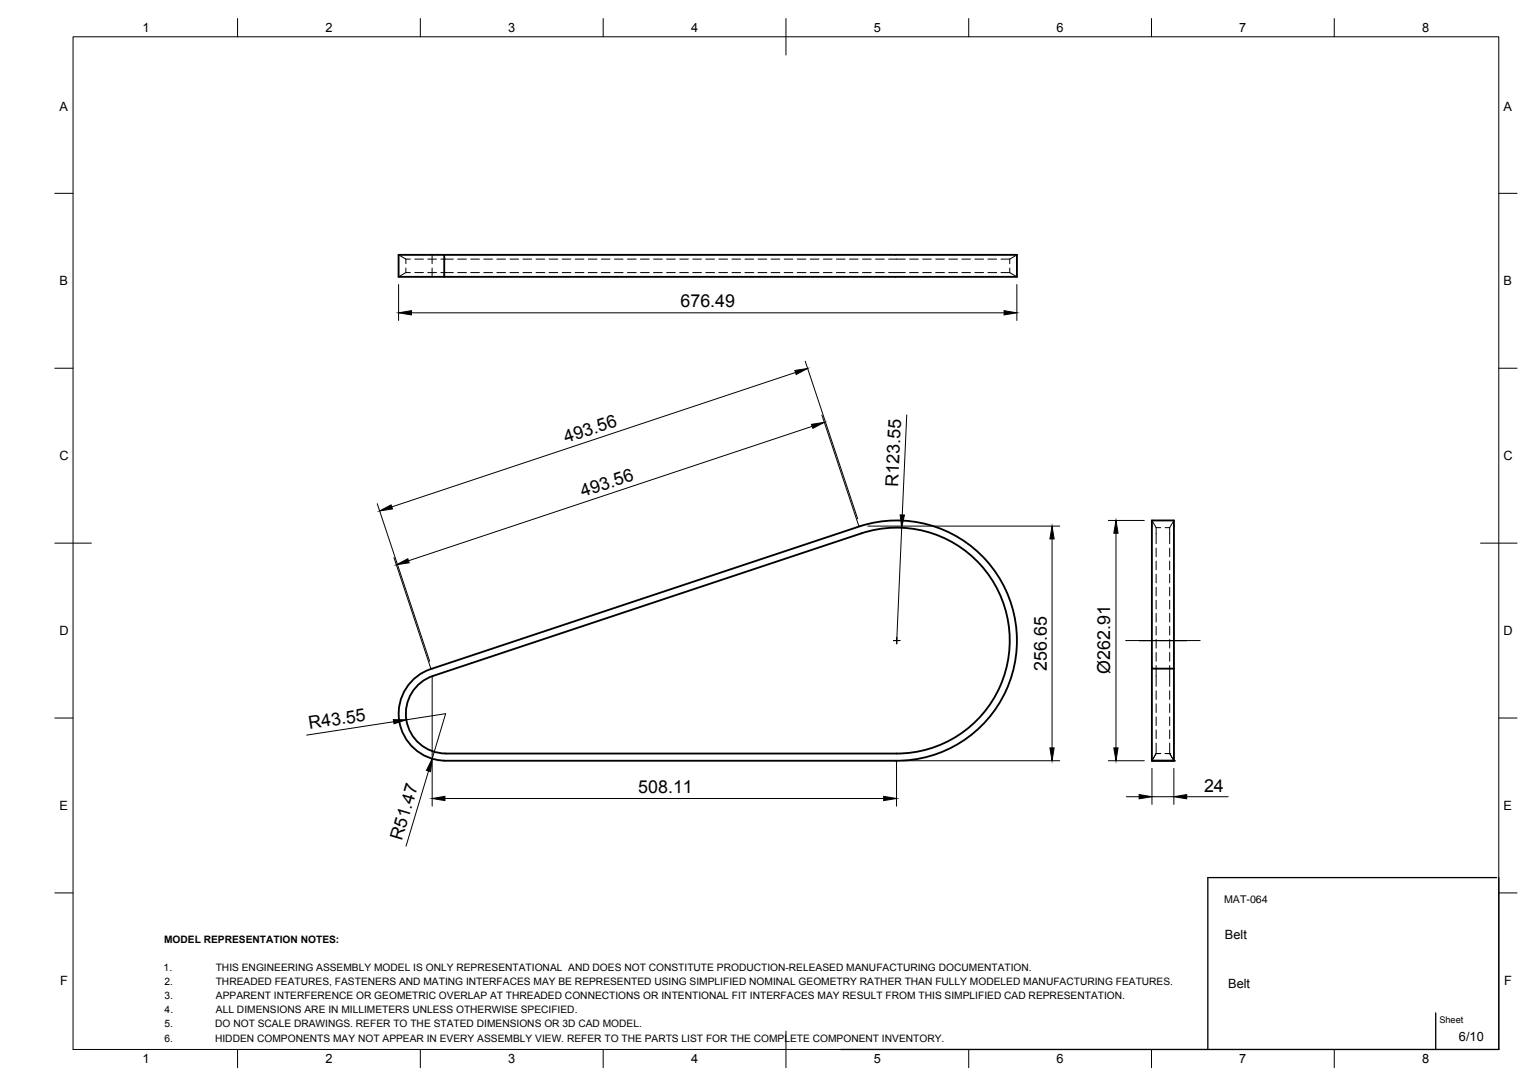
ISO-10303-21;
HEADER;
/* Generated by software containing ST-Developer
 * from STEP Tools, Inc. (www.steptools.com) 
 */

FILE_DESCRIPTION(
/* description */ (''),
/* implementation_level */ '2;1');

FILE_NAME(
/* name */ 
'Belt.step',
/* time_stamp */ '2026-10-24T12:42:14-07:00',
/* author */ (''),
/* organization */ (''),
/* preprocessor_version */ 'ST-DEVELOPER v20.2',
/* originating_system */ 'Autodesk Translation Framework v15.15.0.0',
/* authorisation */ '');

FILE_SCHEMA (('AUTOMOTIVE_DESIGN { 1 0 10303 214 3 1 1 }'));
ENDSEC;

DATA;
#10=MECHANICAL_DESIGN_GEOMETRIC_PRESENTATION_REPRESENTATION('',(#71),#6789);
#11=(
BOUNDED_SURFACE()
B_SPLINE_SURFACE(1,3,((#6689,#6690,#6691,#6692),(#6693,#6694,#6695,#6696)),
 .UNSPECIFIED.,.F.,.F.,.F.)
B_SPLINE_SURFACE_WITH_KNOTS((2,2),(4,4),(0.,1.),(0.,1.),.UNSPECIFIED.)
GEOMETRIC_REPRESENTATION_ITEM()
RATIONAL_B_SPLINE_SURFACE(((1.,0.44,0.44,1.),(1.,0.44,0.44,1.)))
REPRESENTATION_ITEM('')
SURFACE()
);
#12=(
BOUNDED_SURFACE()
B_SPLINE_SURFACE(1,3,((#6704,#6705,#6706,#6707),(#6708,#6709,#6710,#6711)),
 .UNSPECIFIED.,.F.,.F.,.F.)
B_SPLINE_SURFACE_WITH_KNOTS((2,2),(4,4),(0.,1.),(0.,1.),.UNSPECIFIED.)
GEOMETRIC_REPRESENTATION_ITEM()
RATIONAL_B_SPLINE_SURFACE(((1.,0.44,0.44,1.),(1.,0.44,0.44,1.)))
REPRESENTATION_ITEM('')
SURFACE()
);
#13=(
BOUNDED_SURFACE()
B_SPLINE_SURFACE(1,3,((#6733,#6734,#6735,#6736,#6737,#6738,#6739),(#6740,
#6741,#6742,#6743,#6744,#6745,#6746)),.UNSPECIFIED.,.F.,.F.,.F.)
B_SPLINE_SURFACE_WITH_KNOTS((2,2),(4,3,4),(0.,1.),(0.,0.5,1.),
 .UNSPECIFIED.)
GEOMETRIC_REPRESENTATION_ITEM()
RATIONAL_B_SPLINE_SURFACE(((1.,0.765382713227191,0.765382713227191,1.,0.765382713227191,
0.765382713227191,1.),(1.,0.765382713227191,0.765382713227191,1.,0.765382713227191,
0.765382713227191,1.)))
REPRESENTATION_ITEM('')
SURFACE()
);
#14=(
BOUNDED_SURFACE()
B_SPLINE_SURFACE(1,3,((#6750,#6751,#6752,#6753,#6754,#6755,#6756),(#6757,
#6758,#6759,#6760,#6761,#6762,#6763)),.UNSPECIFIED.,.F.,.F.,.F.)
B_SPLINE_SURFACE_WITH_KNOTS((2,2),(4,3,4),(0.,1.),(0.,0.5,1.),
 .UNSPECIFIED.)
GEOMETRIC_REPRESENTATION_ITEM()
RATIONAL_B_SPLINE_SURFACE(((1.,0.765382713227191,0.765382713227191,1.,0.765382713227191,
0.765382713227191,1.),(1.,0.765382713227191,0.765382713227191,1.,0.765382713227191,
0.765382713227191,1.)))
REPRESENTATION_ITEM('')
SURFACE()
);
#59=SHAPE_REPRESENTATION_RELATIONSHIP('SRR','None',#6826,#65);
#65=ADVANCED_BREP_SHAPE_REPRESENTATION('',(#77),#6788);
#71=STYLED_ITEM('',(#6863),#77);
#77=MANIFOLD_SOLID_BREP('Belt',#3966);
#181=CYLINDRICAL_SURFACE('',#4409,51.471200702168);
#182=CYLINDRICAL_SURFACE('',#4413,43.5522017822105);
#183=CYLINDRICAL_SURFACE('',#4419,131.457333002004);
#184=CYLINDRICAL_SURFACE('',#4423,123.55173167544);
#386=CIRCLE('',#4410,51.471200702168);
#387=CIRCLE('',#4411,51.471200702168);
#388=CIRCLE('',#4412,43.5522017822105);
#389=CIRCLE('',#4414,43.5522017822105);
#390=CIRCLE('',#4420,131.457333002004);
#391=CIRCLE('',#4421,131.457333002004);
#392=CIRCLE('',#4422,123.55173167544);
#393=CIRCLE('',#4424,123.55173167544);
#595=FACE_OUTER_BOUND('',#869,.T.);
#596=FACE_OUTER_BOUND('',#870,.T.);
#597=FACE_OUTER_BOUND('',#871,.T.);
#598=FACE_OUTER_BOUND('',#872,.T.);
#599=FACE_OUTER_BOUND('',#873,.T.);
#600=FACE_OUTER_BOUND('',#874,.T.);
#601=FACE_OUTER_BOUND('',#875,.T.);
#602=FACE_OUTER_BOUND('',#876,.T.);
#603=FACE_OUTER_BOUND('',#877,.T.);
#604=FACE_OUTER_BOUND('',#878,.T.);
#605=FACE_OUTER_BOUND('',#879,.T.);
#606=FACE_OUTER_BOUND('',#880,.T.);
#607=FACE_OUTER_BOUND('',#881,.T.);
#608=FACE_OUTER_BOUND('',#882,.T.);
#609=FACE_OUTER_BOUND('',#883,.T.);
#610=FACE_OUTER_BOUND('',#884,.T.);
#869=EDGE_LOOP('',(#3561,#3562,#3563,#3564));
#870=EDGE_LOOP('',(#3565,#3566,#3567,#3568));
#871=EDGE_LOOP('',(#3569,#3570,#3571,#3572));
#872=EDGE_LOOP('',(#3573,#3574,#3575,#3576));
#873=EDGE_LOOP('',(#3577,#3578,#3579,#3580));
#874=EDGE_LOOP('',(#3581,#3582,#3583,#3584));
#875=EDGE_LOOP('',(#3585,#3586,#3587,#3588));
#876=EDGE_LOOP('',(#3589,#3590,#3591,#3592));
#877=EDGE_LOOP('',(#3593,#3594,#3595,#3596));
#878=EDGE_LOOP('',(#3597,#3598,#3599,#3600));
#879=EDGE_LOOP('',(#3601,#3602,#3603,#3604));
#880=EDGE_LOOP('',(#3605,#3606,#3607,#3608));
#881=EDGE_LOOP('',(#3609,#3610,#3611,#3612));
#882=EDGE_LOOP('',(#3613,#3614,#3615,#3616));
#883=EDGE_LOOP('',(#3617,#3618,#3619,#3620));
#884=EDGE_LOOP('',(#3621,#3622,#3623,#3624));
#1239=LINE('',#6665,#1617);
#1240=LINE('',#6667,#1618);
#1241=LINE('',#6669,#1619);
#1242=LINE('',#6670,#1620);
#1243=LINE('',#6674,#1621);
#1244=LINE('',#6675,#1622);
#1245=LINE('',#6676,#1623);
#1246=LINE('',#6680,#1624);
#1247=LINE('',#6681,#1625);
#1248=LINE('',#6682,#1626);
#1249=LINE('',#6687,#1627);
#1250=LINE('',#6699,#1628);
#1251=LINE('',#6703,#1629);
#1252=LINE('',#6712,#1630);
#1253=LINE('',#6713,#1631);
#1254=LINE('',#6716,#1632);
#1255=LINE('',#6718,#1633);
#1256=LINE('',#6719,#1634);
#1257=LINE('',#6722,#1635);
#1258=LINE('',#6723,#1636);
#1259=LINE('',#6726,#1637);
#1260=LINE('',#6727,#1638);
#1261=LINE('',#6729,#1639);
#1262=LINE('',#6764,#1640);
#1617=VECTOR('',#5532,493.558507170122);
#1618=VECTOR('',#5533,24.);
#1619=VECTOR('',#5534,493.558507170122);
#1620=VECTOR('',#5535,24.);
#1621=VECTOR('',#5538,493.558507170122);
#1622=VECTOR('',#5539,9.23760430703403);
#1623=VECTOR('',#5540,9.23760430703403);
#1624=VECTOR('',#5543,493.558507170122);
#1625=VECTOR('',#5544,14.762395692966);
#1626=VECTOR('',#5545,14.762395692966);
#1627=VECTOR('',#5550,24.);
#1628=VECTOR('',#5555,9.23760430703401);
#1629=VECTOR('',#5560,14.762395692966);
#1630=VECTOR('',#5561,9.237604307034);
#1631=VECTOR('',#5562,9.23760430703398);
#1632=VECTOR('',#5565,493.558507170122);
#1633=VECTOR('',#5566,24.);
#1634=VECTOR('',#5567,493.558507170122);
#1635=VECTOR('',#5570,493.558507170122);
#1636=VECTOR('',#5571,9.23760430703404);
#1637=VECTOR('',#5574,493.558507170122);
#1638=VECTOR('',#5575,14.762395692966);
#1639=VECTOR('',#5578,9.237604307034);
#1640=VECTOR('',#5591,9.23760430703399);
#1971=VERTEX_POINT('',#6663);
#1972=VERTEX_POINT('',#6664);
#1973=VERTEX_POINT('',#6666);
#1974=VERTEX_POINT('',#6668);
#1975=VERTEX_POINT('',#6672);
#1976=VERTEX_POINT('',#6673);
#1977=VERTEX_POINT('',#6678);
#1978=VERTEX_POINT('',#6679);
#1979=VERTEX_POINT('',#6684);
#1980=VERTEX_POINT('',#6686);
#1981=VERTEX_POINT('',#6697);
#1982=VERTEX_POINT('',#6701);
#1983=VERTEX_POINT('',#6715);
#1984=VERTEX_POINT('',#6717);
#1985=VERTEX_POINT('',#6721);
#1986=VERTEX_POINT('',#6725);
#2501=EDGE_CURVE('',#1971,#1972,#1239,.T.);
#2502=EDGE_CURVE('',#1971,#1973,#1240,.T.);
#2503=EDGE_CURVE('',#1973,#1974,#1241,.T.);
#2504=EDGE_CURVE('',#1972,#1974,#1242,.T.);
#2505=EDGE_CURVE('',#1975,#1976,#1243,.T.);
#2506=EDGE_CURVE('',#1975,#1971,#1244,.T.);
#2507=EDGE_CURVE('',#1976,#1972,#1245,.T.);
#2508=EDGE_CURVE('',#1977,#1978,#1246,.T.);
#2509=EDGE_CURVE('',#1977,#1975,#1247,.T.);
#2510=EDGE_CURVE('',#1978,#1976,#1248,.T.);
#2511=EDGE_CURVE('',#1979,#1971,#386,.T.);
#2512=EDGE_CURVE('',#1979,#1980,#1249,.T.);
#2513=EDGE_CURVE('',#1980,#1973,#387,.T.);
#2514=EDGE_CURVE('',#1981,#1975,#388,.T.);
#2515=EDGE_CURVE('',#1981,#1979,#1250,.T.);
#2516=EDGE_CURVE('',#1982,#1977,#389,.T.);
#2517=EDGE_CURVE('',#1982,#1981,#1251,.T.);
#2518=EDGE_CURVE('',#1973,#1977,#1252,.T.);
#2519=EDGE_CURVE('',#1980,#1982,#1253,.T.);
#2520=EDGE_CURVE('',#1983,#1979,#1254,.T.);
#2521=EDGE_CURVE('',#1983,#1984,#1255,.T.);
#2522=EDGE_CURVE('',#1984,#1980,#1256,.T.);
#2523=EDGE_CURVE('',#1985,#1981,#1257,.T.);
#2524=EDGE_CURVE('',#1985,#1983,#1258,.T.);
#2525=EDGE_CURVE('',#1986,#1982,#1259,.T.);
#2526=EDGE_CURVE('',#1986,#1985,#1260,.T.);
#2527=EDGE_CURVE('',#1984,#1986,#1261,.T.);
#2528=EDGE_CURVE('',#1972,#1983,#390,.T.);
#2529=EDGE_CURVE('',#1974,#1984,#391,.T.);
#2530=EDGE_CURVE('',#1976,#1985,#392,.T.);
#2531=EDGE_CURVE('',#1978,#1986,#393,.T.);
#2532=EDGE_CURVE('',#1974,#1978,#1262,.T.);
#3561=ORIENTED_EDGE('',*,*,#2501,.F.);
#3562=ORIENTED_EDGE('',*,*,#2502,.T.);
#3563=ORIENTED_EDGE('',*,*,#2503,.T.);
#3564=ORIENTED_EDGE('',*,*,#2504,.F.);
#3565=ORIENTED_EDGE('',*,*,#2505,.F.);
#3566=ORIENTED_EDGE('',*,*,#2506,.T.);
#3567=ORIENTED_EDGE('',*,*,#2501,.T.);
#3568=ORIENTED_EDGE('',*,*,#2507,.F.);
#3569=ORIENTED_EDGE('',*,*,#2508,.F.);
#3570=ORIENTED_EDGE('',*,*,#2509,.T.);
#3571=ORIENTED_EDGE('',*,*,#2505,.T.);
#3572=ORIENTED_EDGE('',*,*,#2510,.F.);
#3573=ORIENTED_EDGE('',*,*,#2502,.F.);
#3574=ORIENTED_EDGE('',*,*,#2511,.F.);
#3575=ORIENTED_EDGE('',*,*,#2512,.T.);
#3576=ORIENTED_EDGE('',*,*,#2513,.T.);
#3577=ORIENTED_EDGE('',*,*,#2511,.T.);
#3578=ORIENTED_EDGE('',*,*,#2506,.F.);
#3579=ORIENTED_EDGE('',*,*,#2514,.F.);
#3580=ORIENTED_EDGE('',*,*,#2515,.T.);
#3581=ORIENTED_EDGE('',*,*,#2514,.T.);
#3582=ORIENTED_EDGE('',*,*,#2509,.F.);
#3583=ORIENTED_EDGE('',*,*,#2516,.F.);
#3584=ORIENTED_EDGE('',*,*,#2517,.T.);
#3585=ORIENTED_EDGE('',*,*,#2516,.T.);
#3586=ORIENTED_EDGE('',*,*,#2518,.F.);
#3587=ORIENTED_EDGE('',*,*,#2513,.F.);
#3588=ORIENTED_EDGE('',*,*,#2519,.T.);
#3589=ORIENTED_EDGE('',*,*,#2512,.F.);
#3590=ORIENTED_EDGE('',*,*,#2520,.F.);
#3591=ORIENTED_EDGE('',*,*,#2521,.T.);
#3592=ORIENTED_EDGE('',*,*,#2522,.T.);
#3593=ORIENTED_EDGE('',*,*,#2520,.T.);
#3594=ORIENTED_EDGE('',*,*,#2515,.F.);
#3595=ORIENTED_EDGE('',*,*,#2523,.F.);
#3596=ORIENTED_EDGE('',*,*,#2524,.T.);
#3597=ORIENTED_EDGE('',*,*,#2523,.T.);
#3598=ORIENTED_EDGE('',*,*,#2517,.F.);
#3599=ORIENTED_EDGE('',*,*,#2525,.F.);
#3600=ORIENTED_EDGE('',*,*,#2526,.T.);
#3601=ORIENTED_EDGE('',*,*,#2525,.T.);
#3602=ORIENTED_EDGE('',*,*,#2519,.F.);
#3603=ORIENTED_EDGE('',*,*,#2522,.F.);
#3604=ORIENTED_EDGE('',*,*,#2527,.T.);
#3605=ORIENTED_EDGE('',*,*,#2521,.F.);
#3606=ORIENTED_EDGE('',*,*,#2528,.F.);
#3607=ORIENTED_EDGE('',*,*,#2504,.T.);
#3608=ORIENTED_EDGE('',*,*,#2529,.T.);
#3609=ORIENTED_EDGE('',*,*,#2528,.T.);
#3610=ORIENTED_EDGE('',*,*,#2524,.F.);
#3611=ORIENTED_EDGE('',*,*,#2530,.F.);
#3612=ORIENTED_EDGE('',*,*,#2507,.T.);
#3613=ORIENTED_EDGE('',*,*,#2530,.T.);
#3614=ORIENTED_EDGE('',*,*,#2526,.F.);
#3615=ORIENTED_EDGE('',*,*,#2531,.F.);
#3616=ORIENTED_EDGE('',*,*,#2510,.T.);
#3617=ORIENTED_EDGE('',*,*,#2531,.T.);
#3618=ORIENTED_EDGE('',*,*,#2527,.F.);
#3619=ORIENTED_EDGE('',*,*,#2529,.F.);
#3620=ORIENTED_EDGE('',*,*,#2532,.T.);
#3621=ORIENTED_EDGE('',*,*,#2518,.T.);
#3622=ORIENTED_EDGE('',*,*,#2508,.T.);
#3623=ORIENTED_EDGE('',*,*,#2532,.F.);
#3624=ORIENTED_EDGE('',*,*,#2503,.F.);
#3736=PLANE('',#4406);
#3737=PLANE('',#4407);
#3738=PLANE('',#4408);
#3739=PLANE('',#4415);
#3740=PLANE('',#4416);
#3741=PLANE('',#4417);
#3742=PLANE('',#4418);
#3743=PLANE('',#4425);
#3945=ADVANCED_FACE('',(#595),#3736,.T.);
#3946=ADVANCED_FACE('',(#596),#3737,.T.);
#3947=ADVANCED_FACE('',(#597),#3738,.T.);
#3948=ADVANCED_FACE('',(#598),#181,.T.);
#3949=ADVANCED_FACE('',(#599),#11,.T.);
#3950=ADVANCED_FACE('',(#600),#182,.F.);
#3951=ADVANCED_FACE('',(#601),#12,.T.);
#3952=ADVANCED_FACE('',(#602),#3739,.T.);
#3953=ADVANCED_FACE('',(#603),#3740,.T.);
#3954=ADVANCED_FACE('',(#604),#3741,.T.);
#3955=ADVANCED_FACE('',(#605),#3742,.T.);
#3956=ADVANCED_FACE('',(#606),#183,.T.);
#3957=ADVANCED_FACE('',(#607),#13,.T.);
#3958=ADVANCED_FACE('',(#608),#184,.F.);
#3959=ADVANCED_FACE('',(#609),#14,.T.);
#3960=ADVANCED_FACE('',(#610),#3743,.T.);
#3966=CLOSED_SHELL('',(#3945,#3946,#3947,#3948,#3949,#3950,#3951,#3952,
#3953,#3954,#3955,#3956,#3957,#3958,#3959,#3960));
#4405=AXIS2_PLACEMENT_3D('',#6661,#5528,#5529);
#4406=AXIS2_PLACEMENT_3D('',#6662,#5530,#5531);
#4407=AXIS2_PLACEMENT_3D('',#6671,#5536,#5537);
#4408=AXIS2_PLACEMENT_3D('',#6677,#5541,#5542);
#4409=AXIS2_PLACEMENT_3D('',#6683,#5546,#5547);
#4410=AXIS2_PLACEMENT_3D('',#6685,#5548,#5549);
#4411=AXIS2_PLACEMENT_3D('',#6688,#5551,#5552);
#4412=AXIS2_PLACEMENT_3D('',#6698,#5553,#5554);
#4413=AXIS2_PLACEMENT_3D('',#6700,#5556,#5557);
#4414=AXIS2_PLACEMENT_3D('',#6702,#5558,#5559);
#4415=AXIS2_PLACEMENT_3D('',#6714,#5563,#5564);
#4416=AXIS2_PLACEMENT_3D('',#6720,#5568,#5569);
#4417=AXIS2_PLACEMENT_3D('',#6724,#5572,#5573);
#4418=AXIS2_PLACEMENT_3D('',#6728,#5576,#5577);
#4419=AXIS2_PLACEMENT_3D('',#6730,#5579,#5580);
#4420=AXIS2_PLACEMENT_3D('',#6731,#5581,#5582);
#4421=AXIS2_PLACEMENT_3D('',#6732,#5583,#5584);
#4422=AXIS2_PLACEMENT_3D('',#6747,#5585,#5586);
#4423=AXIS2_PLACEMENT_3D('',#6748,#5587,#5588);
#4424=AXIS2_PLACEMENT_3D('',#6749,#5589,#5590);
#4425=AXIS2_PLACEMENT_3D('',#6765,#5592,#5593);
#5528=DIRECTION('axis',(0.,0.,1.));
#5529=DIRECTION('refdir',(1.,0.,0.));
#5530=DIRECTION('center_axis',(-0.159999999999998,0.987117014340246,0.));
#5531=DIRECTION('ref_axis',(0.,0.,1.));
#5532=DIRECTION('',(0.987117014340246,0.159999999999998,0.));
#5533=DIRECTION('',(0.,0.,1.));
#5534=DIRECTION('',(0.987117014340246,0.159999999999998,0.));
#5535=DIRECTION('',(0.,0.,1.));
#5536=DIRECTION('center_axis',(0.0807792391722015,-0.498366008702133,-0.863195247837398));
#5537=DIRECTION('ref_axis',(-0.995649789053195,0.,-0.0931745542427157));
#5538=DIRECTION('',(0.987117014340246,0.159999999999998,0.));
#5539=DIRECTION('',(0.,0.866025403784436,-0.500000000000004));
#5540=DIRECTION('',(0.,0.866025403784436,-0.500000000000004));
#5541=DIRECTION('center_axis',(0.159999999999998,-0.987117014340246,0.));
#5542=DIRECTION('ref_axis',(0.,0.,-1.));
#5543=DIRECTION('',(0.987117014340246,0.159999999999998,0.));
#5544=DIRECTION('',(0.,0.,-1.));
#5545=DIRECTION('',(0.,0.,-1.));
#5546=DIRECTION('center_axis',(0.,0.,-1.));
#5547=DIRECTION('ref_axis',(-1.,0.,0.));
#5548=DIRECTION('center_axis',(0.,0.,-1.));
#5549=DIRECTION('ref_axis',(-0.189299873786385,-0.98191932346016,0.));
#5550=DIRECTION('',(0.,0.,1.));
#5551=DIRECTION('center_axis',(0.,0.,-1.));
#5552=DIRECTION('ref_axis',(-0.189299873786385,-0.98191932346016,0.));
#5553=DIRECTION('center_axis',(0.,0.,-1.));
#5554=DIRECTION('ref_axis',(-0.1656970702866,-0.986176698618679,0.));
#5555=DIRECTION('',(-0.273557891496469,-0.821684903110675,-0.500000000000006));
#5556=DIRECTION('center_axis',(0.,0.,-1.));
#5557=DIRECTION('ref_axis',(-1.,0.,0.));
#5558=DIRECTION('center_axis',(0.,0.,-1.));
#5559=DIRECTION('ref_axis',(-0.1656970702866,-0.986176698618679,0.));
#5560=DIRECTION('',(0.,0.,-1.));
#5561=DIRECTION('',(0.,-0.86602540378444,-0.499999999999998));
#5562=DIRECTION('',(0.27355789149647,0.821684903110679,-0.5));
#5563=DIRECTION('center_axis',(-0.160000000000002,-0.987117014340245,0.));
#5564=DIRECTION('ref_axis',(0.,0.,-1.));
#5565=DIRECTION('',(-0.987117014340245,0.160000000000002,0.));
#5566=DIRECTION('',(0.,0.,1.));
#5567=DIRECTION('',(-0.987117014340245,0.160000000000002,0.));
#5568=DIRECTION('center_axis',(0.0807792391722037,0.498366008702132,-0.863195247837398));
#5569=DIRECTION('ref_axis',(-0.995649789053195,0.,-0.0931745542427182));
#5570=DIRECTION('',(-0.987117014340245,0.160000000000002,0.));
#5571=DIRECTION('',(-0.273557891496479,-0.821684903110674,-0.500000000000003));
#5572=DIRECTION('center_axis',(0.160000000000002,0.987117014340245,0.));
#5573=DIRECTION('ref_axis',(0.,0.,1.));
#5574=DIRECTION('',(-0.987117014340245,0.160000000000002,0.));
#5575=DIRECTION('',(0.,0.,-1.));
#5576=DIRECTION('center_axis',(0.0807792391722028,0.498366008702126,0.863195247837401));
#5577=DIRECTION('ref_axis',(0.995649789053195,0.,-0.0931745542427167));
#5578=DIRECTION('',(0.27355789149648,0.821684903110677,-0.499999999999997));
#5579=DIRECTION('center_axis',(0.,0.,-1.));
#5580=DIRECTION('ref_axis',(0.999932136628903,-0.0116499844101919,0.));
#5581=DIRECTION('center_axis',(0.,0.,-1.));
#5582=DIRECTION('ref_axis',(-0.148489244032527,0.988914022757615,0.));
#5583=DIRECTION('center_axis',(0.,0.,-1.));
#5584=DIRECTION('ref_axis',(-0.148489244032527,0.988914022757615,0.));
#5585=DIRECTION('center_axis',(0.,0.,-1.));
#5586=DIRECTION('ref_axis',(-0.157990501106671,0.987440631916706,0.));
#5587=DIRECTION('center_axis',(0.,0.,-1.));
#5588=DIRECTION('ref_axis',(0.999997928592931,-0.00203538936013715,0.));
#5589=DIRECTION('center_axis',(0.,0.,-1.));
#5590=DIRECTION('ref_axis',(-0.157990501106671,0.987440631916706,0.));
#5591=DIRECTION('',(0.,-0.86602540378444,-0.499999999999998));
#5592=DIRECTION('center_axis',(0.0807792391722006,-0.498366008702127,0.863195247837401));
#5593=DIRECTION('ref_axis',(0.995649789053195,0.,-0.0931745542427143));
#6661=CARTESIAN_POINT('',(0.,0.,0.));
#6662=CARTESIAN_POINT('Origin',(-506.719999999999,51.0306388527815,12.));
#6663=CARTESIAN_POINT('',(-506.719999999999,51.0306388527815,-12.));
#6664=CARTESIAN_POINT('',(-19.5199999999996,130.,-12.));
#6665=CARTESIAN_POINT('',(-506.719999999999,51.0306388527815,-12.));
#6666=CARTESIAN_POINT('',(-506.719999999999,51.0306388527815,12.));
#6667=CARTESIAN_POINT('',(-506.719999999999,51.0306388527815,-12.));
#6668=CARTESIAN_POINT('',(-19.5199999999996,130.,12.));
#6669=CARTESIAN_POINT('',(-506.719999999999,51.0306388527815,12.));
#6670=CARTESIAN_POINT('',(-19.5199999999996,130.,-12.));
#6671=CARTESIAN_POINT('Origin',(-506.719999999999,51.0306388527815,-12.));
#6672=CARTESIAN_POINT('',(-506.719999999999,43.0306388527815,-7.38119784648294));
#6673=CARTESIAN_POINT('',(-19.5199999999996,122.,-7.38119784648294));
#6674=CARTESIAN_POINT('',(-506.719999999999,43.0306388527815,-7.38119784648294));
#6675=CARTESIAN_POINT('',(-506.719999999999,43.0306388527815,-7.38119784648295));
#6676=CARTESIAN_POINT('',(-19.5199999999996,122.,-7.38119784648295));
#6677=CARTESIAN_POINT('Origin',(-506.719999999999,43.0306388527815,7.38119784648301));
#6678=CARTESIAN_POINT('',(-506.719999999999,43.0306388527815,7.38119784648301));
#6679=CARTESIAN_POINT('',(-19.5199999999996,122.,7.38119784648301));
#6680=CARTESIAN_POINT('',(-506.719999999999,43.0306388527815,7.38119784648301));
#6681=CARTESIAN_POINT('',(-506.719999999999,43.0306388527815,7.38119784648301));
#6682=CARTESIAN_POINT('',(-19.5199999999996,122.,7.38119784648301));
#6683=CARTESIAN_POINT('Origin',(-499.999999999999,1.45487256761396E-12,
0.));
#6684=CARTESIAN_POINT('',(-509.743491796554,-50.5405665711541,-12.));
#6685=CARTESIAN_POINT('Origin',(-499.999999999999,1.45487256761396E-12,
-12.));
#6686=CARTESIAN_POINT('',(-509.743491796554,-50.5405665711541,12.));
#6687=CARTESIAN_POINT('',(-509.743491796554,-50.5405665711534,-12.));
#6688=CARTESIAN_POINT('Origin',(-499.999999999999,1.45487256761396E-12,
12.));
#6689=CARTESIAN_POINT('Ctrl Pts',(-507.216472239843,-42.9501665711535,-7.38119784648294));
#6690=CARTESIAN_POINT('Ctrl Pts',(-571.454108893077,-32.1569809174214,-7.38119784648294));
#6691=CARTESIAN_POINT('Ctrl Pts',(-571.077993559862,32.97999288859,-7.38119784648294));
#6692=CARTESIAN_POINT('Ctrl Pts',(-506.719999999999,43.0306388527815,-7.38119784648294));
#6693=CARTESIAN_POINT('Ctrl Pts',(-509.743491796554,-50.5405665711535,-12.));
#6694=CARTESIAN_POINT('Ctrl Pts',(-585.333572367437,-35.9678900083305,-12.));
#6695=CARTESIAN_POINT('Ctrl Pts',(-583.043048279138,40.9799928885899,-12.));
#6696=CARTESIAN_POINT('Ctrl Pts',(-506.719999999999,51.0306388527815,-12.));
#6697=CARTESIAN_POINT('',(-507.216472239843,-42.9501665711541,-7.38119784648294));
#6698=CARTESIAN_POINT('Origin',(-499.999999999999,1.45487256761396E-12,
-7.38119784648294));
#6699=CARTESIAN_POINT('',(-507.216472239843,-42.9501665711539,-7.38119784648324));
#6700=CARTESIAN_POINT('Origin',(-499.999999999999,1.45487256761396E-12,
0.));
#6701=CARTESIAN_POINT('',(-507.216472239843,-42.9501665711541,7.38119784648301));
#6702=CARTESIAN_POINT('Origin',(-499.999999999999,1.45487256761396E-12,
7.38119784648301));
#6703=CARTESIAN_POINT('',(-507.216472239843,-42.9501665711534,7.38119784648301));
#6704=CARTESIAN_POINT('Ctrl Pts',(-509.743491796554,-50.5405665711535,12.));
#6705=CARTESIAN_POINT('Ctrl Pts',(-585.333572367437,-35.9678900083305,12.));
#6706=CARTESIAN_POINT('Ctrl Pts',(-583.043048279138,40.9799928885899,12.));
#6707=CARTESIAN_POINT('Ctrl Pts',(-506.719999999999,51.0306388527815,12.));
#6708=CARTESIAN_POINT('Ctrl Pts',(-507.216472239843,-42.9501665711535,7.38119784648301));
#6709=CARTESIAN_POINT('Ctrl Pts',(-571.454108893077,-32.1569809174214,7.38119784648301));
#6710=CARTESIAN_POINT('Ctrl Pts',(-571.077993559862,32.97999288859,7.38119784648301));
#6711=CARTESIAN_POINT('Ctrl Pts',(-506.719999999999,43.0306388527815,7.38119784648301));
#6712=CARTESIAN_POINT('',(-506.719999999999,51.0306388527815,12.));
#6713=CARTESIAN_POINT('',(-509.743491796554,-50.5405665711539,12.0000000000003));
#6714=CARTESIAN_POINT('Origin',(-22.5434917965546,-129.509927718375,12.));
#6715=CARTESIAN_POINT('',(-22.5434917965544,-129.509927718374,-12.));
#6716=CARTESIAN_POINT('',(-22.5434917965545,-129.509927718375,-12.));
#6717=CARTESIAN_POINT('',(-22.5434917965544,-129.509927718374,12.));
#6718=CARTESIAN_POINT('',(-22.5434917965546,-129.509927718375,-12.));
#6719=CARTESIAN_POINT('',(-22.5434917965545,-129.509927718375,12.));
#6720=CARTESIAN_POINT('Origin',(-22.5434917965546,-129.509927718375,-12.));
#6721=CARTESIAN_POINT('',(-20.0164722398434,-121.919527718374,-7.38119784648294));
#6722=CARTESIAN_POINT('',(-20.0164722398435,-121.919527718375,-7.38119784648294));
#6723=CARTESIAN_POINT('',(-20.0164722398434,-121.919527718374,-7.38119784648264));
#6724=CARTESIAN_POINT('Origin',(-20.0164722398436,-121.919527718375,7.38119784648301));
#6725=CARTESIAN_POINT('',(-20.0164722398434,-121.919527718374,7.38119784648301));
#6726=CARTESIAN_POINT('',(-20.0164722398435,-121.919527718375,7.38119784648301));
#6727=CARTESIAN_POINT('',(-20.0164722398436,-121.919527718375,7.38119784648301));
#6728=CARTESIAN_POINT('Origin',(-22.5434917965546,-129.509927718375,12.));
#6729=CARTESIAN_POINT('',(-22.5434917965544,-129.509927718374,11.9999999999997));
#6730=CARTESIAN_POINT('Origin',(1.66533453693773E-13,3.77520255149252E-13,
0.));
#6731=CARTESIAN_POINT('Origin',(1.66533453693773E-13,3.77520255149252E-13,
-12.));
#6732=CARTESIAN_POINT('Origin',(1.66533453693773E-13,3.77520255149252E-13,
12.));
#6733=CARTESIAN_POINT('Ctrl Pts',(-19.5199999999996,122.,-7.38119784648294));
#6734=CARTESIAN_POINT('Ctrl Pts',(61.4089525234421,134.948632403751,-7.38119784648294));
#6735=CARTESIAN_POINT('Ctrl Pts',(123.718292795081,81.706651293145,-7.38119784648294));
#6736=CARTESIAN_POINT('Ctrl Pts',(123.55147574951,-0.251475880078228,-7.38119784648294));
#6737=CARTESIAN_POINT('Ctrl Pts',(123.384658703939,-82.2096030533015,-7.38119784648294));
#6738=CARTESIAN_POINT('Ctrl Pts',(60.8590988290158,-135.197496010055,-7.38119784648294));
#6739=CARTESIAN_POINT('Ctrl Pts',(-20.0164722398431,-121.919527718374,-7.38119784648294));
#6740=CARTESIAN_POINT('Ctrl Pts',(-19.5199999999996,130.,-12.));
#6741=CARTESIAN_POINT('Ctrl Pts',(66.7157690823563,142.948632403751,-12.));
#6742=CARTESIAN_POINT('Ctrl Pts',(132.464319559229,85.6651002104318,-12.));
#6743=CARTESIAN_POINT('Ctrl Pts',(131.448411864232,-1.53147588007823,-12.));
#6744=CARTESIAN_POINT('Ctrl Pts',(130.432504169234,-88.7280519705883,-12.));
#6745=CARTESIAN_POINT('Ctrl Pts',(63.3671868234026,-144.464199663587,-12.));
#6746=CARTESIAN_POINT('Ctrl Pts',(-22.5434917965542,-129.509927718374,-12.));
#6747=CARTESIAN_POINT('Origin',(1.66533453693773E-13,3.77520255149252E-13,
-7.38119784648294));
#6748=CARTESIAN_POINT('Origin',(1.66533453693773E-13,3.77520255149252E-13,
0.));
#6749=CARTESIAN_POINT('Origin',(1.66533453693773E-13,3.77520255149252E-13,
7.38119784648301));
#6750=CARTESIAN_POINT('Ctrl Pts',(-19.5199999999996,130.,12.));
#6751=CARTESIAN_POINT('Ctrl Pts',(66.7157690823563,142.948632403751,12.));
#6752=CARTESIAN_POINT('Ctrl Pts',(132.464319559229,85.6651002104318,12.));
#6753=CARTESIAN_POINT('Ctrl Pts',(131.448411864232,-1.53147588007823,12.));
#6754=CARTESIAN_POINT('Ctrl Pts',(130.432504169234,-88.7280519705883,12.));
#6755=CARTESIAN_POINT('Ctrl Pts',(63.3671868234026,-144.464199663587,12.));
#6756=CARTESIAN_POINT('Ctrl Pts',(-22.5434917965542,-129.509927718374,12.));
#6757=CARTESIAN_POINT('Ctrl Pts',(-19.5199999999996,122.,7.38119784648301));
#6758=CARTESIAN_POINT('Ctrl Pts',(61.4089525234421,134.948632403751,7.38119784648302));
#6759=CARTESIAN_POINT('Ctrl Pts',(123.718292795081,81.706651293145,7.38119784648302));
#6760=CARTESIAN_POINT('Ctrl Pts',(123.55147574951,-0.251475880078228,7.38119784648301));
#6761=CARTESIAN_POINT('Ctrl Pts',(123.384658703939,-82.2096030533015,7.38119784648302));
#6762=CARTESIAN_POINT('Ctrl Pts',(60.8590988290158,-135.197496010055,7.38119784648302));
#6763=CARTESIAN_POINT('Ctrl Pts',(-20.0164722398431,-121.919527718374,7.38119784648301));
#6764=CARTESIAN_POINT('',(-19.5199999999996,130.,12.));
#6765=CARTESIAN_POINT('Origin',(-506.719999999999,51.0306388527815,12.));
#6779=UNCERTAINTY_MEASURE_WITH_UNIT(LENGTH_MEASURE(0.01),#6790,
'DISTANCE_ACCURACY_VALUE',
'Maximum model space distance between geometric entities at asserted c
onnectivities');
#6780=UNCERTAINTY_MEASURE_WITH_UNIT(LENGTH_MEASURE(0.01),#6790,
'DISTANCE_ACCURACY_VALUE',
'Maximum model space distance between geometric entities at asserted c
onnectivities');
#6788=(
GEOMETRIC_REPRESENTATION_CONTEXT(3)
GLOBAL_UNCERTAINTY_ASSIGNED_CONTEXT((#6779))
GLOBAL_UNIT_ASSIGNED_CONTEXT((#6790,#6792,#6793))
REPRESENTATION_CONTEXT('','3D')
);
#6789=(
GEOMETRIC_REPRESENTATION_CONTEXT(3)
GLOBAL_UNCERTAINTY_ASSIGNED_CONTEXT((#6780))
GLOBAL_UNIT_ASSIGNED_CONTEXT((#6790,#6792,#6793))
REPRESENTATION_CONTEXT('','3D')
);
#6790=(
LENGTH_UNIT()
NAMED_UNIT(*)
SI_UNIT(.MILLI.,.METRE.)
);
#6792=(
NAMED_UNIT(*)
PLANE_ANGLE_UNIT()
SI_UNIT($,.RADIAN.)
);
#6793=(
NAMED_UNIT(*)
SI_UNIT($,.STERADIAN.)
SOLID_ANGLE_UNIT()
);
#6801=SHAPE_DEFINITION_REPRESENTATION(#6812,#6826);
#6812=PRODUCT_DEFINITION_SHAPE('',$,#6835);
#6826=SHAPE_REPRESENTATION('',(#4405),#6788);
#6827=PRODUCT_DEFINITION_CONTEXT('part definition',#6853,'design');
#6835=PRODUCT_DEFINITION('Belt','Belt',#6843,#6827);
#6843=PRODUCT_DEFINITION_FORMATION('',$,#6862);
#6853=APPLICATION_CONTEXT(
'Core Data for Automotive Mechanical Design Process');
#6854=PRODUCT_CONTEXT('part definition',#6853,'mechanical');
#6862=PRODUCT('Belt','Belt','Belt1-13__ DE    13309',(#6854));
#6863=PRESENTATION_STYLE_ASSIGNMENT((#6865));
#6865=SURFACE_STYLE_USAGE(.BOTH.,#6867);
#6867=SURFACE_SIDE_STYLE('',(#6869));
#6869=SURFACE_STYLE_FILL_AREA(#6871);
#6871=FILL_AREA_STYLE('Steel - Satin',(#6873));
#6873=FILL_AREA_STYLE_COLOUR('Steel - Satin',#6875);
#6875=COLOUR_RGB('Steel - Satin',0.627450980392157,0.627450980392157,0.627450980392157);
ENDSEC;
END-ISO-10303-21;
